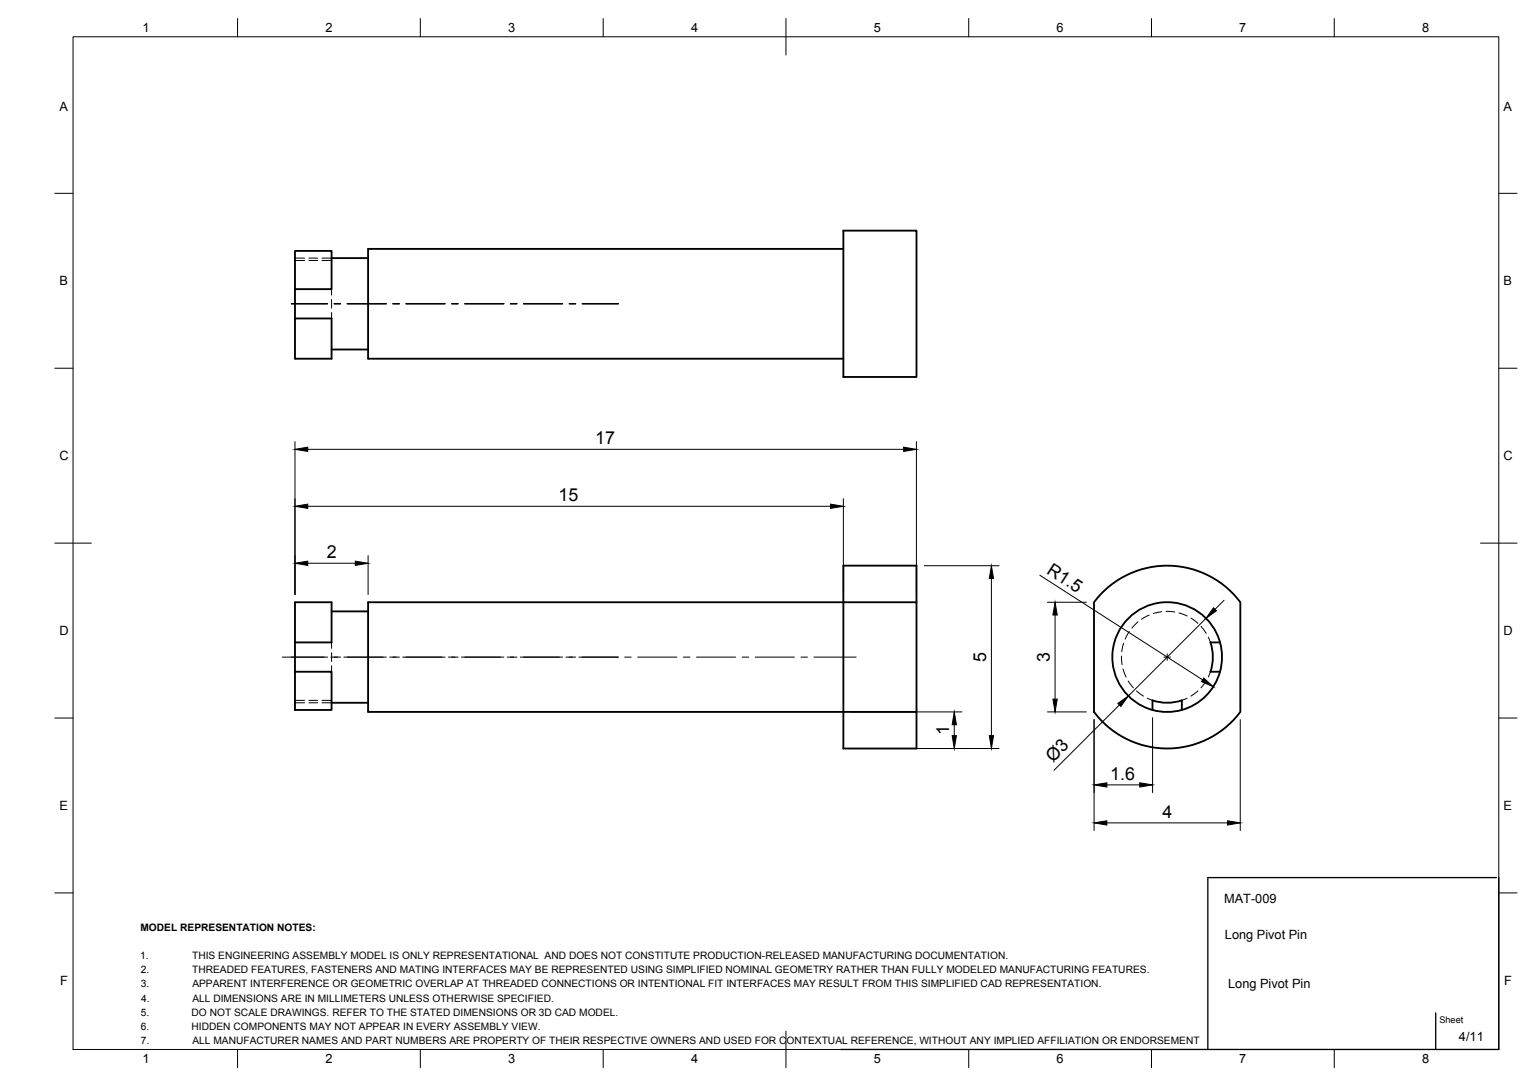
ISO-10303-21;
HEADER;
/* Generated by software containing ST-Developer
 * from STEP Tools, Inc. (www.steptools.com) 
 */

FILE_DESCRIPTION(
/* description */ ('STEP AP214'),
/* implementation_level */ '2;1');

FILE_NAME(
/* name */ 'Long Pivot Pin.step',
/* time_stamp */ '2026-11-14T05:43:09-08:00',
/* author */ (''),
/* organization */ (''),
/* preprocessor_version */ 'ST-DEVELOPER v20.2',
/* originating_system */ 'Autodesk Translation Framework v15.17.0.0',
/* authorisation */ '');

FILE_SCHEMA (('AUTOMOTIVE_DESIGN { 1 0 10303 214 3 1 1 }'));
ENDSEC;

DATA;
#10=MECHANICAL_DESIGN_GEOMETRIC_PRESENTATION_REPRESENTATION('',(#151),#11933);
#133=SHAPE_REPRESENTATION_RELATIONSHIP('SRR','None',#11993,#142);
#142=ADVANCED_BREP_SHAPE_REPRESENTATION('',(#160),#11929);
#151=STYLED_ITEM('',(#12042),#160);
#160=MANIFOLD_SOLID_BREP('Body1',#6648);
#198=FACE_BOUND('',#998,.T.);
#199=FACE_BOUND('',#1000,.T.);
#276=PLANE('',#7497);
#277=PLANE('',#7501);
#278=PLANE('',#7502);
#279=PLANE('',#7507);
#280=PLANE('',#7510);
#281=PLANE('',#7511);
#282=PLANE('',#7512);
#283=PLANE('',#7516);
#284=PLANE('',#7517);
#285=PLANE('',#7518);
#286=PLANE('',#7519);
#287=PLANE('',#7520);
#605=FACE_OUTER_BOUND('',#993,.T.);
#606=FACE_OUTER_BOUND('',#994,.T.);
#607=FACE_OUTER_BOUND('',#995,.T.);
#608=FACE_OUTER_BOUND('',#996,.T.);
#609=FACE_OUTER_BOUND('',#997,.T.);
#610=FACE_OUTER_BOUND('',#999,.T.);
#611=FACE_OUTER_BOUND('',#1001,.T.);
#612=FACE_OUTER_BOUND('',#1002,.T.);
#613=FACE_OUTER_BOUND('',#1003,.T.);
#614=FACE_OUTER_BOUND('',#1004,.T.);
#615=FACE_OUTER_BOUND('',#1005,.T.);
#616=FACE_OUTER_BOUND('',#1006,.T.);
#617=FACE_OUTER_BOUND('',#1007,.T.);
#618=FACE_OUTER_BOUND('',#1008,.T.);
#619=FACE_OUTER_BOUND('',#1009,.T.);
#620=FACE_OUTER_BOUND('',#1010,.T.);
#621=FACE_OUTER_BOUND('',#1011,.T.);
#622=FACE_OUTER_BOUND('',#1012,.T.);
#993=EDGE_LOOP('',(#5728,#5729,#5730,#5731,#5732,#5733,#5734,#5735,#5736,
#5737,#5738,#5739));
#994=EDGE_LOOP('',(#5740,#5741,#5742,#5743));
#995=EDGE_LOOP('',(#5744,#5745,#5746,#5747));
#996=EDGE_LOOP('',(#5748,#5749,#5750,#5751));
#997=EDGE_LOOP('',(#5752));
#998=EDGE_LOOP('',(#5753));
#999=EDGE_LOOP('',(#5754,#5755,#5756,#5757));
#1000=EDGE_LOOP('',(#5758));
#1001=EDGE_LOOP('',(#5759,#5760,#5761,#5762));
#1002=EDGE_LOOP('',(#5763,#5764,#5765,#5766));
#1003=EDGE_LOOP('',(#5767,#5768,#5769,#5770));
#1004=EDGE_LOOP('',(#5771,#5772,#5773,#5774));
#1005=EDGE_LOOP('',(#5775,#5776,#5777,#5778));
#1006=EDGE_LOOP('',(#5779,#5780,#5781,#5782,#5783));
#1007=EDGE_LOOP('',(#5784,#5785,#5786,#5787));
#1008=EDGE_LOOP('',(#5788,#5789,#5790,#5791,#5792,#5793,#5794,#5795));
#1009=EDGE_LOOP('',(#5796,#5797,#5798,#5799));
#1010=EDGE_LOOP('',(#5800,#5801,#5802,#5803));
#1011=EDGE_LOOP('',(#5804,#5805,#5806,#5807));
#1012=EDGE_LOOP('',(#5808,#5809,#5810,#5811));
#1438=LINE('',#11551,#1900);
#1439=LINE('',#11555,#1901);
#1440=LINE('',#11559,#1902);
#1441=LINE('',#11563,#1903);
#1442=LINE('',#11567,#1904);
#1443=LINE('',#11573,#1905);
#1444=LINE('',#11577,#1906);
#1445=LINE('',#11580,#1907);
#1446=LINE('',#11583,#1908);
#1447=LINE('',#11586,#1909);
#1448=LINE('',#11593,#1910);
#1449=LINE('',#11596,#1911);
#1450=LINE('',#11601,#1912);
#1451=LINE('',#11602,#1913);
#1452=LINE('',#11605,#1914);
#1453=LINE('',#11606,#1915);
#1454=LINE('',#11610,#1916);
#1455=LINE('',#11612,#1917);
#1456=LINE('',#11618,#1918);
#1457=LINE('',#11619,#1919);
#1458=LINE('',#11624,#1920);
#1459=LINE('',#11625,#1921);
#1460=LINE('',#11627,#1922);
#1461=LINE('',#11628,#1923);
#1462=LINE('',#11629,#1924);
#1463=LINE('',#11630,#1925);
#1900=VECTOR('',#9490,1.25);
#1901=VECTOR('',#9493,1000.);
#1902=VECTOR('',#9496,1000.);
#1903=VECTOR('',#9499,1000.);
#1904=VECTOR('',#9502,1000.);
#1905=VECTOR('',#9509,1.5);
#1906=VECTOR('',#9514,1000.);
#1907=VECTOR('',#9517,1000.);
#1908=VECTOR('',#9520,1000.);
#1909=VECTOR('',#9523,1000.);
#1910=VECTOR('',#9530,1000.);
#1911=VECTOR('',#9533,1000.);
#1912=VECTOR('',#9538,1000.);
#1913=VECTOR('',#9539,1000.);
#1914=VECTOR('',#9542,1000.);
#1915=VECTOR('',#9543,1000.);
#1916=VECTOR('',#9548,1000.);
#1917=VECTOR('',#9551,1000.);
#1918=VECTOR('',#9558,1000.);
#1919=VECTOR('',#9559,1000.);
#1920=VECTOR('',#9564,1000.);
#1921=VECTOR('',#9565,1000.);
#1922=VECTOR('',#9568,1000.);
#1923=VECTOR('',#9569,1000.);
#1924=VECTOR('',#9570,1000.);
#1925=VECTOR('',#9571,1000.);
#2438=CIRCLE('',#7488,1.25);
#2439=CIRCLE('',#7489,1.25);
#2440=CIRCLE('',#7490,1.25);
#2441=CIRCLE('',#7491,1.25);
#2442=CIRCLE('',#7492,1.25);
#2443=CIRCLE('',#7493,1.25);
#2444=CIRCLE('',#7495,1.5);
#2445=CIRCLE('',#7496,1.5);
#2446=CIRCLE('',#7498,1.5);
#2447=CIRCLE('',#7500,1.5);
#2448=CIRCLE('',#7503,2.5);
#2449=CIRCLE('',#7504,2.5);
#2450=CIRCLE('',#7506,2.5);
#2451=CIRCLE('',#7509,2.5);
#2452=CIRCLE('',#7513,1.5);
#2453=CIRCLE('',#7515,1.5);
#3039=VERTEX_POINT('',#11548);
#3040=VERTEX_POINT('',#11550);
#3041=VERTEX_POINT('',#11552);
#3042=VERTEX_POINT('',#11554);
#3043=VERTEX_POINT('',#11556);
#3044=VERTEX_POINT('',#11558);
#3045=VERTEX_POINT('',#11560);
#3046=VERTEX_POINT('',#11562);
#3047=VERTEX_POINT('',#11564);
#3048=VERTEX_POINT('',#11566);
#3049=VERTEX_POINT('',#11570);
#3050=VERTEX_POINT('',#11572);
#3051=VERTEX_POINT('',#11576);
#3052=VERTEX_POINT('',#11578);
#3053=VERTEX_POINT('',#11582);
#3054=VERTEX_POINT('',#11584);
#3055=VERTEX_POINT('',#11589);
#3056=VERTEX_POINT('',#11590);
#3057=VERTEX_POINT('',#11592);
#3058=VERTEX_POINT('',#11594);
#3059=VERTEX_POINT('',#11598);
#3060=VERTEX_POINT('',#11599);
#3061=VERTEX_POINT('',#11604);
#3062=VERTEX_POINT('',#11608);
#3063=VERTEX_POINT('',#11615);
#3064=VERTEX_POINT('',#11616);
#3065=VERTEX_POINT('',#11621);
#3066=VERTEX_POINT('',#11622);
#3953=EDGE_CURVE('',#3039,#3039,#2438,.T.);
#3954=EDGE_CURVE('',#3039,#3040,#1438,.T.);
#3955=EDGE_CURVE('',#3041,#3040,#2439,.T.);
#3956=EDGE_CURVE('',#3041,#3042,#1439,.T.);
#3957=EDGE_CURVE('',#3042,#3043,#2440,.T.);
#3958=EDGE_CURVE('',#3044,#3043,#1440,.T.);
#3959=EDGE_CURVE('',#3045,#3044,#2441,.T.);
#3960=EDGE_CURVE('',#3045,#3046,#1441,.T.);
#3961=EDGE_CURVE('',#3046,#3047,#2442,.T.);
#3962=EDGE_CURVE('',#3048,#3047,#1442,.T.);
#3963=EDGE_CURVE('',#3040,#3048,#2443,.T.);
#3964=EDGE_CURVE('',#3049,#3049,#2444,.T.);
#3965=EDGE_CURVE('',#3049,#3050,#1443,.T.);
#3966=EDGE_CURVE('',#3050,#3050,#2445,.T.);
#3967=EDGE_CURVE('',#3044,#3051,#1444,.T.);
#3968=EDGE_CURVE('',#3052,#3051,#2446,.T.);
#3969=EDGE_CURVE('',#3052,#3045,#1445,.T.);
#3970=EDGE_CURVE('',#3051,#3053,#1446,.T.);
#3971=EDGE_CURVE('',#3054,#3053,#2447,.T.);
#3972=EDGE_CURVE('',#3052,#3054,#1447,.T.);
#3973=EDGE_CURVE('',#3055,#3056,#2448,.T.);
#3974=EDGE_CURVE('',#3056,#3057,#1448,.T.);
#3975=EDGE_CURVE('',#3057,#3058,#2449,.T.);
#3976=EDGE_CURVE('',#3058,#3055,#1449,.T.);
#3977=EDGE_CURVE('',#3059,#3060,#2450,.T.);
#3978=EDGE_CURVE('',#3056,#3060,#1450,.T.);
#3979=EDGE_CURVE('',#3055,#3059,#1451,.T.);
#3980=EDGE_CURVE('',#3060,#3061,#1452,.T.);
#3981=EDGE_CURVE('',#3057,#3061,#1453,.T.);
#3982=EDGE_CURVE('',#3061,#3062,#2451,.T.);
#3983=EDGE_CURVE('',#3058,#3062,#1454,.T.);
#3984=EDGE_CURVE('',#3062,#3059,#1455,.T.);
#3985=EDGE_CURVE('',#3063,#3064,#2452,.T.);
#3986=EDGE_CURVE('',#3063,#3041,#1456,.T.);
#3987=EDGE_CURVE('',#3048,#3064,#1457,.T.);
#3988=EDGE_CURVE('',#3065,#3066,#2453,.T.);
#3989=EDGE_CURVE('',#3063,#3065,#1458,.T.);
#3990=EDGE_CURVE('',#3064,#3066,#1459,.T.);
#3991=EDGE_CURVE('',#3043,#3053,#1460,.T.);
#3992=EDGE_CURVE('',#3065,#3042,#1461,.T.);
#3993=EDGE_CURVE('',#3047,#3066,#1462,.T.);
#3994=EDGE_CURVE('',#3054,#3046,#1463,.T.);
#5728=ORIENTED_EDGE('',*,*,#3953,.T.);
#5729=ORIENTED_EDGE('',*,*,#3954,.T.);
#5730=ORIENTED_EDGE('',*,*,#3955,.F.);
#5731=ORIENTED_EDGE('',*,*,#3956,.T.);
#5732=ORIENTED_EDGE('',*,*,#3957,.T.);
#5733=ORIENTED_EDGE('',*,*,#3958,.F.);
#5734=ORIENTED_EDGE('',*,*,#3959,.F.);
#5735=ORIENTED_EDGE('',*,*,#3960,.T.);
#5736=ORIENTED_EDGE('',*,*,#3961,.T.);
#5737=ORIENTED_EDGE('',*,*,#3962,.F.);
#5738=ORIENTED_EDGE('',*,*,#3963,.F.);
#5739=ORIENTED_EDGE('',*,*,#3954,.F.);
#5740=ORIENTED_EDGE('',*,*,#3964,.T.);
#5741=ORIENTED_EDGE('',*,*,#3965,.T.);
#5742=ORIENTED_EDGE('',*,*,#3966,.F.);
#5743=ORIENTED_EDGE('',*,*,#3965,.F.);
#5744=ORIENTED_EDGE('',*,*,#3959,.T.);
#5745=ORIENTED_EDGE('',*,*,#3967,.T.);
#5746=ORIENTED_EDGE('',*,*,#3968,.F.);
#5747=ORIENTED_EDGE('',*,*,#3969,.T.);
#5748=ORIENTED_EDGE('',*,*,#3968,.T.);
#5749=ORIENTED_EDGE('',*,*,#3970,.T.);
#5750=ORIENTED_EDGE('',*,*,#3971,.F.);
#5751=ORIENTED_EDGE('',*,*,#3972,.F.);
#5752=ORIENTED_EDGE('',*,*,#3966,.T.);
#5753=ORIENTED_EDGE('',*,*,#3953,.F.);
#5754=ORIENTED_EDGE('',*,*,#3973,.T.);
#5755=ORIENTED_EDGE('',*,*,#3974,.T.);
#5756=ORIENTED_EDGE('',*,*,#3975,.T.);
#5757=ORIENTED_EDGE('',*,*,#3976,.T.);
#5758=ORIENTED_EDGE('',*,*,#3964,.F.);
#5759=ORIENTED_EDGE('',*,*,#3977,.T.);
#5760=ORIENTED_EDGE('',*,*,#3978,.F.);
#5761=ORIENTED_EDGE('',*,*,#3973,.F.);
#5762=ORIENTED_EDGE('',*,*,#3979,.T.);
#5763=ORIENTED_EDGE('',*,*,#3980,.T.);
#5764=ORIENTED_EDGE('',*,*,#3981,.F.);
#5765=ORIENTED_EDGE('',*,*,#3974,.F.);
#5766=ORIENTED_EDGE('',*,*,#3978,.T.);
#5767=ORIENTED_EDGE('',*,*,#3982,.T.);
#5768=ORIENTED_EDGE('',*,*,#3983,.F.);
#5769=ORIENTED_EDGE('',*,*,#3975,.F.);
#5770=ORIENTED_EDGE('',*,*,#3981,.T.);
#5771=ORIENTED_EDGE('',*,*,#3984,.T.);
#5772=ORIENTED_EDGE('',*,*,#3979,.F.);
#5773=ORIENTED_EDGE('',*,*,#3976,.F.);
#5774=ORIENTED_EDGE('',*,*,#3983,.T.);
#5775=ORIENTED_EDGE('',*,*,#3977,.F.);
#5776=ORIENTED_EDGE('',*,*,#3984,.F.);
#5777=ORIENTED_EDGE('',*,*,#3982,.F.);
#5778=ORIENTED_EDGE('',*,*,#3980,.F.);
#5779=ORIENTED_EDGE('',*,*,#3985,.F.);
#5780=ORIENTED_EDGE('',*,*,#3986,.T.);
#5781=ORIENTED_EDGE('',*,*,#3955,.T.);
#5782=ORIENTED_EDGE('',*,*,#3963,.T.);
#5783=ORIENTED_EDGE('',*,*,#3987,.T.);
#5784=ORIENTED_EDGE('',*,*,#3988,.F.);
#5785=ORIENTED_EDGE('',*,*,#3989,.F.);
#5786=ORIENTED_EDGE('',*,*,#3985,.T.);
#5787=ORIENTED_EDGE('',*,*,#3990,.T.);
#5788=ORIENTED_EDGE('',*,*,#3991,.F.);
#5789=ORIENTED_EDGE('',*,*,#3957,.F.);
#5790=ORIENTED_EDGE('',*,*,#3992,.F.);
#5791=ORIENTED_EDGE('',*,*,#3988,.T.);
#5792=ORIENTED_EDGE('',*,*,#3993,.F.);
#5793=ORIENTED_EDGE('',*,*,#3961,.F.);
#5794=ORIENTED_EDGE('',*,*,#3994,.F.);
#5795=ORIENTED_EDGE('',*,*,#3971,.T.);
#5796=ORIENTED_EDGE('',*,*,#3993,.T.);
#5797=ORIENTED_EDGE('',*,*,#3990,.F.);
#5798=ORIENTED_EDGE('',*,*,#3987,.F.);
#5799=ORIENTED_EDGE('',*,*,#3962,.T.);
#5800=ORIENTED_EDGE('',*,*,#3994,.T.);
#5801=ORIENTED_EDGE('',*,*,#3960,.F.);
#5802=ORIENTED_EDGE('',*,*,#3969,.F.);
#5803=ORIENTED_EDGE('',*,*,#3972,.T.);
#5804=ORIENTED_EDGE('',*,*,#3991,.T.);
#5805=ORIENTED_EDGE('',*,*,#3970,.F.);
#5806=ORIENTED_EDGE('',*,*,#3967,.F.);
#5807=ORIENTED_EDGE('',*,*,#3958,.T.);
#5808=ORIENTED_EDGE('',*,*,#3992,.T.);
#5809=ORIENTED_EDGE('',*,*,#3956,.F.);
#5810=ORIENTED_EDGE('',*,*,#3986,.F.);
#5811=ORIENTED_EDGE('',*,*,#3989,.T.);
#6265=CYLINDRICAL_SURFACE('',#7487,1.25);
#6266=CYLINDRICAL_SURFACE('',#7494,1.5);
#6267=CYLINDRICAL_SURFACE('',#7499,1.5);
#6268=CYLINDRICAL_SURFACE('',#7505,2.5);
#6269=CYLINDRICAL_SURFACE('',#7508,2.5);
#6270=CYLINDRICAL_SURFACE('',#7514,1.5);
#6575=ADVANCED_FACE('',(#605),#6265,.T.);
#6576=ADVANCED_FACE('',(#606),#6266,.T.);
#6577=ADVANCED_FACE('',(#607),#276,.F.);
#6578=ADVANCED_FACE('',(#608),#6267,.T.);
#6579=ADVANCED_FACE('',(#609,#198),#277,.T.);
#6580=ADVANCED_FACE('',(#610,#199),#278,.T.);
#6581=ADVANCED_FACE('',(#611),#6268,.T.);
#6582=ADVANCED_FACE('',(#612),#279,.F.);
#6583=ADVANCED_FACE('',(#613),#6269,.T.);
#6584=ADVANCED_FACE('',(#614),#280,.F.);
#6585=ADVANCED_FACE('',(#615),#281,.F.);
#6586=ADVANCED_FACE('',(#616),#282,.F.);
#6587=ADVANCED_FACE('',(#617),#6270,.T.);
#6588=ADVANCED_FACE('',(#618),#283,.T.);
#6589=ADVANCED_FACE('',(#619),#284,.F.);
#6590=ADVANCED_FACE('',(#620),#285,.F.);
#6591=ADVANCED_FACE('',(#621),#286,.F.);
#6592=ADVANCED_FACE('',(#622),#287,.F.);
#6648=CLOSED_SHELL('',(#6575,#6576,#6577,#6578,#6579,#6580,#6581,#6582,
#6583,#6584,#6585,#6586,#6587,#6588,#6589,#6590,#6591,#6592));
#7486=AXIS2_PLACEMENT_3D('',#11546,#9484,#9485);
#7487=AXIS2_PLACEMENT_3D('',#11547,#9486,#9487);
#7488=AXIS2_PLACEMENT_3D('',#11549,#9488,#9489);
#7489=AXIS2_PLACEMENT_3D('',#11553,#9491,#9492);
#7490=AXIS2_PLACEMENT_3D('',#11557,#9494,#9495);
#7491=AXIS2_PLACEMENT_3D('',#11561,#9497,#9498);
#7492=AXIS2_PLACEMENT_3D('',#11565,#9500,#9501);
#7493=AXIS2_PLACEMENT_3D('',#11568,#9503,#9504);
#7494=AXIS2_PLACEMENT_3D('',#11569,#9505,#9506);
#7495=AXIS2_PLACEMENT_3D('',#11571,#9507,#9508);
#7496=AXIS2_PLACEMENT_3D('',#11574,#9510,#9511);
#7497=AXIS2_PLACEMENT_3D('',#11575,#9512,#9513);
#7498=AXIS2_PLACEMENT_3D('',#11579,#9515,#9516);
#7499=AXIS2_PLACEMENT_3D('',#11581,#9518,#9519);
#7500=AXIS2_PLACEMENT_3D('',#11585,#9521,#9522);
#7501=AXIS2_PLACEMENT_3D('',#11587,#9524,#9525);
#7502=AXIS2_PLACEMENT_3D('',#11588,#9526,#9527);
#7503=AXIS2_PLACEMENT_3D('',#11591,#9528,#9529);
#7504=AXIS2_PLACEMENT_3D('',#11595,#9531,#9532);
#7505=AXIS2_PLACEMENT_3D('',#11597,#9534,#9535);
#7506=AXIS2_PLACEMENT_3D('',#11600,#9536,#9537);
#7507=AXIS2_PLACEMENT_3D('',#11603,#9540,#9541);
#7508=AXIS2_PLACEMENT_3D('',#11607,#9544,#9545);
#7509=AXIS2_PLACEMENT_3D('',#11609,#9546,#9547);
#7510=AXIS2_PLACEMENT_3D('',#11611,#9549,#9550);
#7511=AXIS2_PLACEMENT_3D('',#11613,#9552,#9553);
#7512=AXIS2_PLACEMENT_3D('',#11614,#9554,#9555);
#7513=AXIS2_PLACEMENT_3D('',#11617,#9556,#9557);
#7514=AXIS2_PLACEMENT_3D('',#11620,#9560,#9561);
#7515=AXIS2_PLACEMENT_3D('',#11623,#9562,#9563);
#7516=AXIS2_PLACEMENT_3D('',#11626,#9566,#9567);
#7517=AXIS2_PLACEMENT_3D('',#11631,#9572,#9573);
#7518=AXIS2_PLACEMENT_3D('',#11632,#9574,#9575);
#7519=AXIS2_PLACEMENT_3D('',#11633,#9576,#9577);
#7520=AXIS2_PLACEMENT_3D('',#11634,#9578,#9579);
#9484=DIRECTION('axis',(0.,0.,1.));
#9485=DIRECTION('refdir',(1.,0.,0.));
#9486=DIRECTION('center_axis',(0.,0.,-1.));
#9487=DIRECTION('ref_axis',(-1.,0.,0.));
#9488=DIRECTION('center_axis',(0.,0.,1.));
#9489=DIRECTION('ref_axis',(1.,0.,0.));
#9490=DIRECTION('',(0.,0.,1.));
#9491=DIRECTION('center_axis',(0.,0.,1.));
#9492=DIRECTION('ref_axis',(1.,0.,0.));
#9493=DIRECTION('',(0.,0.,1.));
#9494=DIRECTION('center_axis',(0.,0.,-1.));
#9495=DIRECTION('ref_axis',(1.,0.,0.));
#9496=DIRECTION('',(0.,0.,1.));
#9497=DIRECTION('center_axis',(0.,0.,1.));
#9498=DIRECTION('ref_axis',(1.,0.,0.));
#9499=DIRECTION('',(0.,0.,1.));
#9500=DIRECTION('center_axis',(0.,0.,-1.));
#9501=DIRECTION('ref_axis',(1.,0.,0.));
#9502=DIRECTION('',(0.,0.,1.));
#9503=DIRECTION('center_axis',(0.,0.,1.));
#9504=DIRECTION('ref_axis',(1.,0.,0.));
#9505=DIRECTION('center_axis',(0.,0.,-1.));
#9506=DIRECTION('ref_axis',(-1.,0.,0.));
#9507=DIRECTION('center_axis',(0.,0.,1.));
#9508=DIRECTION('ref_axis',(1.,0.,0.));
#9509=DIRECTION('',(0.,0.,1.));
#9510=DIRECTION('center_axis',(0.,0.,1.));
#9511=DIRECTION('ref_axis',(1.,0.,0.));
#9512=DIRECTION('center_axis',(0.,0.,1.));
#9513=DIRECTION('ref_axis',(1.,0.,0.));
#9514=DIRECTION('',(-1.,2.07374770584121E-16,0.));
#9515=DIRECTION('center_axis',(0.,0.,1.));
#9516=DIRECTION('ref_axis',(1.,0.,0.));
#9517=DIRECTION('',(2.07374770584121E-16,-1.,0.));
#9518=DIRECTION('center_axis',(0.,0.,-1.));
#9519=DIRECTION('ref_axis',(-1.,0.,0.));
#9520=DIRECTION('',(0.,0.,1.));
#9521=DIRECTION('center_axis',(0.,0.,1.));
#9522=DIRECTION('ref_axis',(1.,0.,0.));
#9523=DIRECTION('',(0.,0.,1.));
#9524=DIRECTION('center_axis',(0.,0.,1.));
#9525=DIRECTION('ref_axis',(1.,0.,0.));
#9526=DIRECTION('center_axis',(0.,0.,1.));
#9527=DIRECTION('ref_axis',(1.,0.,0.));
#9528=DIRECTION('center_axis',(0.,0.,1.));
#9529=DIRECTION('ref_axis',(1.,0.,0.));
#9530=DIRECTION('',(0.,-1.,0.));
#9531=DIRECTION('center_axis',(0.,0.,1.));
#9532=DIRECTION('ref_axis',(1.,0.,0.));
#9533=DIRECTION('',(0.,1.,0.));
#9534=DIRECTION('center_axis',(0.,0.,-1.));
#9535=DIRECTION('ref_axis',(-1.,0.,0.));
#9536=DIRECTION('center_axis',(0.,0.,1.));
#9537=DIRECTION('ref_axis',(1.,0.,0.));
#9538=DIRECTION('',(0.,0.,-1.));
#9539=DIRECTION('',(0.,0.,-1.));
#9540=DIRECTION('center_axis',(1.,0.,0.));
#9541=DIRECTION('ref_axis',(0.,0.,-1.));
#9542=DIRECTION('',(0.,-1.,0.));
#9543=DIRECTION('',(0.,0.,-1.));
#9544=DIRECTION('center_axis',(0.,0.,-1.));
#9545=DIRECTION('ref_axis',(-1.,0.,0.));
#9546=DIRECTION('center_axis',(0.,0.,1.));
#9547=DIRECTION('ref_axis',(1.,0.,0.));
#9548=DIRECTION('',(0.,0.,-1.));
#9549=DIRECTION('center_axis',(-1.,0.,0.));
#9550=DIRECTION('ref_axis',(0.,0.,1.));
#9551=DIRECTION('',(0.,1.,0.));
#9552=DIRECTION('center_axis',(0.,0.,1.));
#9553=DIRECTION('ref_axis',(1.,0.,0.));
#9554=DIRECTION('center_axis',(0.,0.,1.));
#9555=DIRECTION('ref_axis',(1.,0.,0.));
#9556=DIRECTION('center_axis',(0.,0.,1.));
#9557=DIRECTION('ref_axis',(1.,0.,0.));
#9558=DIRECTION('',(1.,2.07374770584121E-16,0.));
#9559=DIRECTION('',(2.07374770584121E-16,1.,0.));
#9560=DIRECTION('center_axis',(0.,0.,-1.));
#9561=DIRECTION('ref_axis',(0.707106781186548,-0.707106781186547,0.));
#9562=DIRECTION('center_axis',(0.,0.,1.));
#9563=DIRECTION('ref_axis',(1.,0.,0.));
#9564=DIRECTION('',(0.,0.,1.));
#9565=DIRECTION('',(0.,0.,1.));
#9566=DIRECTION('center_axis',(0.,0.,1.));
#9567=DIRECTION('ref_axis',(1.,0.,0.));
#9568=DIRECTION('',(-1.,2.07374770584121E-16,0.));
#9569=DIRECTION('',(1.,2.07374770584121E-16,0.));
#9570=DIRECTION('',(2.07374770584121E-16,1.,0.));
#9571=DIRECTION('',(2.07374770584121E-16,-1.,0.));
#9572=DIRECTION('center_axis',(1.,-2.07374770584121E-16,0.));
#9573=DIRECTION('ref_axis',(2.07374770584121E-16,1.,0.));
#9574=DIRECTION('center_axis',(-1.,-2.07374770584121E-16,0.));
#9575=DIRECTION('ref_axis',(2.07374770584121E-16,-1.,0.));
#9576=DIRECTION('center_axis',(2.07374770584121E-16,1.,0.));
#9577=DIRECTION('ref_axis',(-1.,2.07374770584121E-16,0.));
#9578=DIRECTION('center_axis',(2.07374770584121E-16,-1.,0.));
#9579=DIRECTION('ref_axis',(1.,2.07374770584121E-16,0.));
#11546=CARTESIAN_POINT('',(0.,0.,0.));
#11547=CARTESIAN_POINT('Origin',(0.,0.,16.));
#11548=CARTESIAN_POINT('',(1.25,-1.53080849893419E-16,15.));
#11549=CARTESIAN_POINT('Origin',(0.,0.,15.));
#11550=CARTESIAN_POINT('',(1.25,-1.53080849893419E-16,16.));
#11551=CARTESIAN_POINT('',(1.25,-1.53080849893419E-16,16.));
#11552=CARTESIAN_POINT('',(-1.1842719282327,-0.4,16.));
#11553=CARTESIAN_POINT('Origin',(0.,0.,16.));
#11554=CARTESIAN_POINT('',(-1.1842719282327,-0.4,17.));
#11555=CARTESIAN_POINT('',(-1.1842719282327,-0.4,16.));
#11556=CARTESIAN_POINT('',(-1.1842719282327,0.4,17.));
#11557=CARTESIAN_POINT('Origin',(0.,0.,17.));
#11558=CARTESIAN_POINT('',(-1.1842719282327,0.4,16.));
#11559=CARTESIAN_POINT('',(-1.1842719282327,0.4,16.));
#11560=CARTESIAN_POINT('',(-0.4,1.1842719282327,16.));
#11561=CARTESIAN_POINT('Origin',(0.,0.,16.));
#11562=CARTESIAN_POINT('',(-0.4,1.1842719282327,17.));
#11563=CARTESIAN_POINT('',(-0.4,1.1842719282327,16.));
#11564=CARTESIAN_POINT('',(0.4,1.1842719282327,17.));
#11565=CARTESIAN_POINT('Origin',(0.,0.,17.));
#11566=CARTESIAN_POINT('',(0.4,1.1842719282327,16.));
#11567=CARTESIAN_POINT('',(0.4,1.1842719282327,16.));
#11568=CARTESIAN_POINT('Origin',(0.,0.,16.));
#11569=CARTESIAN_POINT('Origin',(0.,0.,15.));
#11570=CARTESIAN_POINT('',(1.5,-1.83697019872103E-16,2.));
#11571=CARTESIAN_POINT('Origin',(0.,0.,2.));
#11572=CARTESIAN_POINT('',(1.5,-1.83697019872103E-16,15.));
#11573=CARTESIAN_POINT('',(1.5,-1.83697019872103E-16,15.));
#11574=CARTESIAN_POINT('Origin',(0.,0.,15.));
#11575=CARTESIAN_POINT('Origin',(0.,0.,16.));
#11576=CARTESIAN_POINT('',(-1.4456832294801,0.4,16.));
#11577=CARTESIAN_POINT('',(-1.1842719282327,0.4,16.));
#11578=CARTESIAN_POINT('',(-0.4,1.4456832294801,16.));
#11579=CARTESIAN_POINT('Origin',(0.,0.,16.));
#11580=CARTESIAN_POINT('',(-0.4,1.1842719282327,16.));
#11581=CARTESIAN_POINT('Origin',(0.,0.,17.));
#11582=CARTESIAN_POINT('',(-1.4456832294801,0.4,17.));
#11583=CARTESIAN_POINT('',(-1.4456832294801,0.4,16.));
#11584=CARTESIAN_POINT('',(-0.4,1.4456832294801,17.));
#11585=CARTESIAN_POINT('Origin',(0.,0.,17.));
#11586=CARTESIAN_POINT('',(-0.4,1.4456832294801,16.));
#11587=CARTESIAN_POINT('Origin',(0.,0.,15.));
#11588=CARTESIAN_POINT('Origin',(0.,0.,2.));
#11589=CARTESIAN_POINT('',(2.,1.5,2.));
#11590=CARTESIAN_POINT('',(-2.,1.5,2.));
#11591=CARTESIAN_POINT('Origin',(0.,0.,2.));
#11592=CARTESIAN_POINT('',(-2.,-1.5,2.));
#11593=CARTESIAN_POINT('',(-2.,1.5,2.));
#11594=CARTESIAN_POINT('',(2.,-1.5,2.));
#11595=CARTESIAN_POINT('Origin',(0.,0.,2.));
#11596=CARTESIAN_POINT('',(2.,1.5,2.));
#11597=CARTESIAN_POINT('Origin',(0.,0.,2.));
#11598=CARTESIAN_POINT('',(2.,1.5,0.));
#11599=CARTESIAN_POINT('',(-2.,1.5,0.));
#11600=CARTESIAN_POINT('Origin',(0.,0.,0.));
#11601=CARTESIAN_POINT('',(-2.,1.5,2.));
#11602=CARTESIAN_POINT('',(2.,1.5,2.));
#11603=CARTESIAN_POINT('Origin',(-2.,1.5,2.));
#11604=CARTESIAN_POINT('',(-2.,-1.5,0.));
#11605=CARTESIAN_POINT('',(-2.,1.5,0.));
#11606=CARTESIAN_POINT('',(-2.,-1.5,2.));
#11607=CARTESIAN_POINT('Origin',(0.,0.,2.));
#11608=CARTESIAN_POINT('',(2.,-1.5,0.));
#11609=CARTESIAN_POINT('Origin',(0.,0.,0.));
#11610=CARTESIAN_POINT('',(2.,-1.5,2.));
#11611=CARTESIAN_POINT('Origin',(2.,1.5,2.));
#11612=CARTESIAN_POINT('',(2.,1.5,0.));
#11613=CARTESIAN_POINT('Origin',(0.,0.,0.));
#11614=CARTESIAN_POINT('Origin',(0.,0.,16.));
#11615=CARTESIAN_POINT('',(-1.4456832294801,-0.4,16.));
#11616=CARTESIAN_POINT('',(0.4,1.4456832294801,16.));
#11617=CARTESIAN_POINT('Origin',(0.,0.,16.));
#11618=CARTESIAN_POINT('',(-1.1842719282327,-0.4,16.));
#11619=CARTESIAN_POINT('',(0.4,1.1842719282327,16.));
#11620=CARTESIAN_POINT('Origin',(0.,0.,17.));
#11621=CARTESIAN_POINT('',(-1.4456832294801,-0.4,17.));
#11622=CARTESIAN_POINT('',(0.4,1.4456832294801,17.));
#11623=CARTESIAN_POINT('Origin',(0.,0.,17.));
#11624=CARTESIAN_POINT('',(-1.4456832294801,-0.4,16.));
#11625=CARTESIAN_POINT('',(0.4,1.4456832294801,16.));
#11626=CARTESIAN_POINT('Origin',(0.,0.,17.));
#11627=CARTESIAN_POINT('',(-1.1842719282327,0.4,17.));
#11628=CARTESIAN_POINT('',(-1.1842719282327,-0.4,17.));
#11629=CARTESIAN_POINT('',(0.4,1.1842719282327,17.));
#11630=CARTESIAN_POINT('',(-0.4,1.1842719282327,17.));
#11631=CARTESIAN_POINT('Origin',(0.4,1.1842719282327,16.));
#11632=CARTESIAN_POINT('Origin',(-0.4,1.1842719282327,16.));
#11633=CARTESIAN_POINT('Origin',(-1.1842719282327,0.4,16.));
#11634=CARTESIAN_POINT('Origin',(-1.1842719282327,-0.4,16.));
#11918=UNCERTAINTY_MEASURE_WITH_UNIT(LENGTH_MEASURE(0.01),#11934,
'DISTANCE_ACCURACY_VALUE',
'Maximum model space distance between geometric entities at asserted c
onnectivities');
#11922=UNCERTAINTY_MEASURE_WITH_UNIT(LENGTH_MEASURE(0.01),#11934,
'DISTANCE_ACCURACY_VALUE',
'Maximum model space distance between geometric entities at asserted c
onnectivities');
#11929=(
GEOMETRIC_REPRESENTATION_CONTEXT(3)
GLOBAL_UNCERTAINTY_ASSIGNED_CONTEXT((#11918))
GLOBAL_UNIT_ASSIGNED_CONTEXT((#11934,#11936,#11937))
REPRESENTATION_CONTEXT('','3D')
);
#11933=(
GEOMETRIC_REPRESENTATION_CONTEXT(3)
GLOBAL_UNCERTAINTY_ASSIGNED_CONTEXT((#11922))
GLOBAL_UNIT_ASSIGNED_CONTEXT((#11934,#11936,#11937))
REPRESENTATION_CONTEXT('','3D')
);
#11934=(
LENGTH_UNIT()
NAMED_UNIT(*)
SI_UNIT(.MILLI.,.METRE.)
);
#11936=(
NAMED_UNIT(*)
PLANE_ANGLE_UNIT()
SI_UNIT($,.RADIAN.)
);
#11937=(
NAMED_UNIT(*)
SI_UNIT($,.STERADIAN.)
SOLID_ANGLE_UNIT()
);
#11944=SHAPE_DEFINITION_REPRESENTATION(#11954,#11993);
#11954=PRODUCT_DEFINITION_SHAPE('',$,#12004);
#11993=SHAPE_REPRESENTATION('',(#7486),#11929);
#11997=PRODUCT_DEFINITION_CONTEXT('part definition',#12029,'design');
#12004=PRODUCT_DEFINITION('Long Pivot Pin','Long Pivot Pin',#12014,#11997);
#12014=PRODUCT_DEFINITION_FORMATION('',$,#12037);
#12029=APPLICATION_CONTEXT(
'Core Data for Automotive Mechanical Design Process');
#12030=PRODUCT_CONTEXT('part definition',#12029,'mechanical');
#12037=PRODUCT('Long Pivot Pin','Long Pivot Pin',$,(#12030));
#12042=PRESENTATION_STYLE_ASSIGNMENT((#12046));
#12046=SURFACE_STYLE_USAGE(.BOTH.,#12050);
#12050=SURFACE_SIDE_STYLE('',(#12054));
#12054=SURFACE_STYLE_FILL_AREA(#12058);
#12058=FILL_AREA_STYLE('Opaque(227,224,212)',(#12062));
#12062=FILL_AREA_STYLE_COLOUR('Opaque(227,224,212)',#12066);
#12066=COLOUR_RGB('Opaque(227,224,212)',0.890196078431372,0.87843137254902,
0.831372549019608);
ENDSEC;
END-ISO-10303-21;
